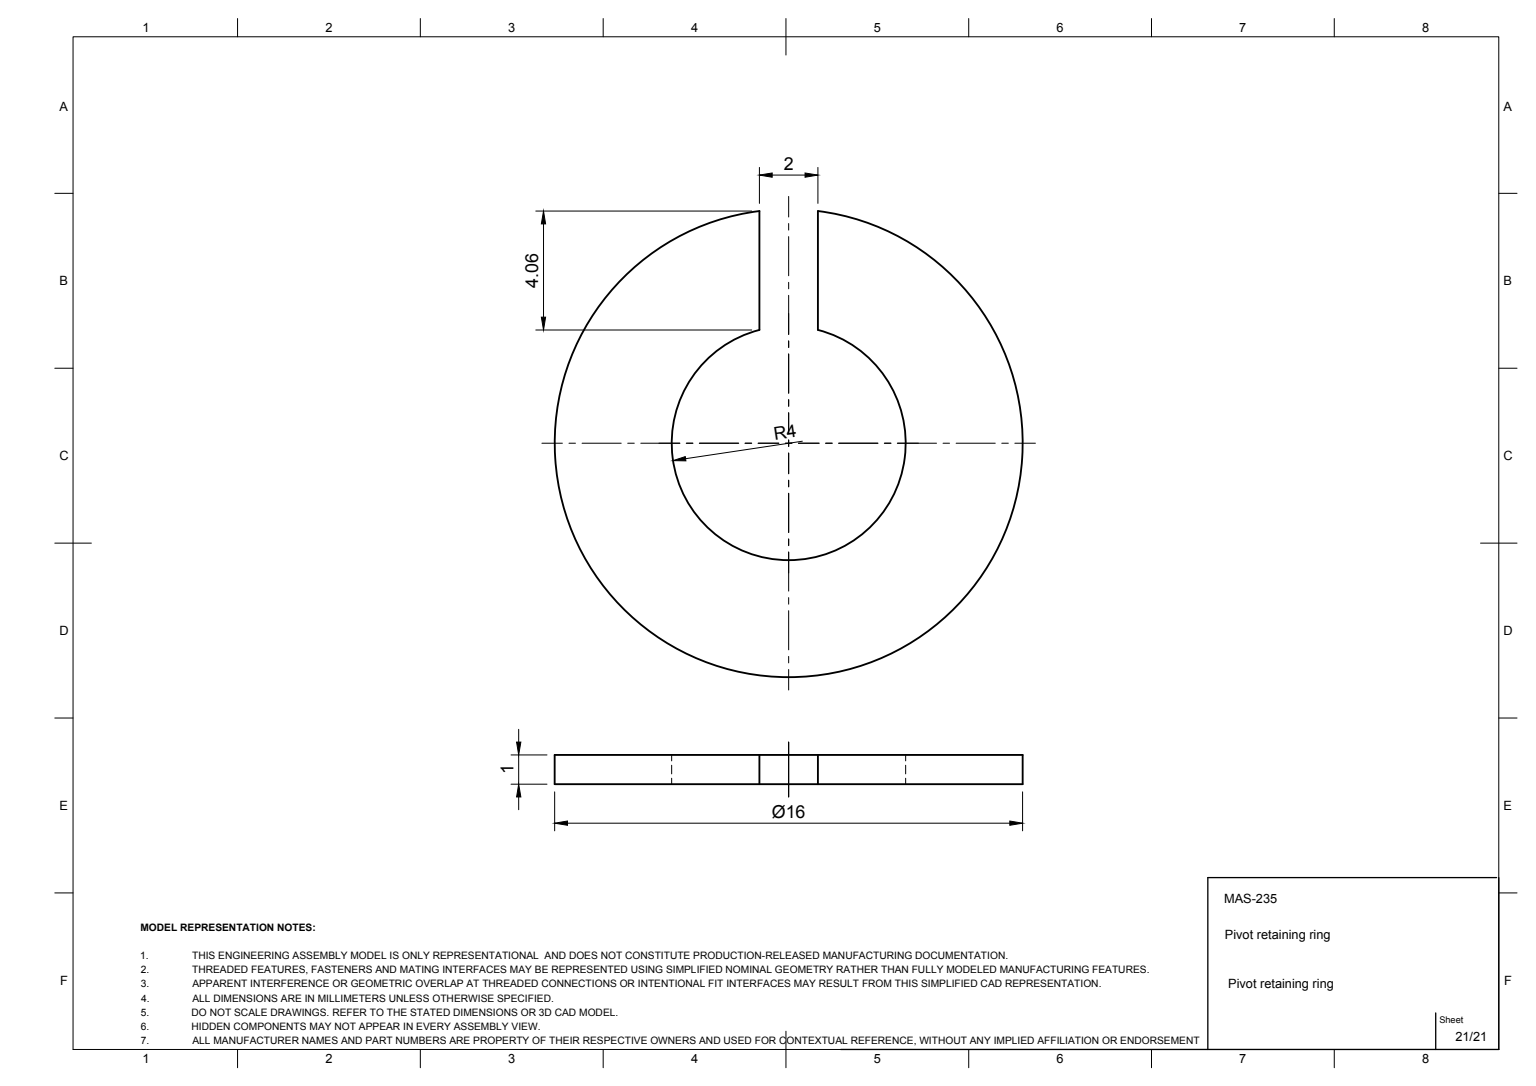
ISO-10303-21;
HEADER;
/* Generated by software containing ST-Developer
 * from STEP Tools, Inc. (www.steptools.com) 
 */

FILE_DESCRIPTION(
/* description */ ('Independent Whitworth quick-return mechanism. Crank radius40, ground-
center spacing80, lever180, connecting rod160, output guide X200. Nomi
nal stroke180 and long/short phase ratio2. Retained guide rods, replac
eable bearing sleeves and captured sliding shoe. No load or production
 rating assigned.'),
/* implementation_level */ '2;1');

FILE_NAME(
/* name */ 'Pivot retaining ring.step',
/* time_stamp */ '2026-11-09T18:22:56-08:00',
/* author */ (''),
/* organization */ (''),
/* preprocessor_version */ 'ST-DEVELOPER v20.2',
/* originating_system */ 'Autodesk Translation Framework v15.17.0.0',
/* authorisation */ '');

FILE_SCHEMA (('AUTOMOTIVE_DESIGN { 1 0 10303 214 3 1 1 }'));
ENDSEC;

DATA;
#10=MECHANICAL_DESIGN_GEOMETRIC_PRESENTATION_REPRESENTATION('',(#238),#4388);
#198=SHAPE_REPRESENTATION_RELATIONSHIP('SRR','None',#4497,#218);
#218=ADVANCED_BREP_SHAPE_REPRESENTATION('',(#258),#4387);
#238=STYLED_ITEM('',(#4599),#258);
#258=MANIFOLD_SOLID_BREP('Body1',#2343);
#401=PLANE('',#2845);
#402=PLANE('',#2846);
#403=PLANE('',#2847);
#404=PLANE('',#2854);
#546=FACE_OUTER_BOUND('',#753,.T.);
#547=FACE_OUTER_BOUND('',#754,.T.);
#548=FACE_OUTER_BOUND('',#755,.T.);
#549=FACE_OUTER_BOUND('',#756,.T.);
#550=FACE_OUTER_BOUND('',#757,.T.);
#551=FACE_OUTER_BOUND('',#758,.T.);
#753=EDGE_LOOP('',(#2092,#2093,#2094,#2095));
#754=EDGE_LOOP('',(#2096,#2097,#2098,#2099));
#755=EDGE_LOOP('',(#2100,#2101,#2102,#2103));
#756=EDGE_LOOP('',(#2104,#2105,#2106,#2107));
#757=EDGE_LOOP('',(#2108,#2109,#2110,#2111));
#758=EDGE_LOOP('',(#2112,#2113,#2114,#2115));
#890=LINE('',#4280,#1029);
#891=LINE('',#4282,#1030);
#892=LINE('',#4284,#1031);
#893=LINE('',#4285,#1032);
#894=LINE('',#4289,#1033);
#895=LINE('',#4291,#1034);
#896=LINE('',#4293,#1035);
#897=LINE('',#4294,#1036);
#1029=VECTOR('',#3590,10.);
#1030=VECTOR('',#3591,10.);
#1031=VECTOR('',#3592,10.);
#1032=VECTOR('',#3593,10.);
#1033=VECTOR('',#3596,10.);
#1034=VECTOR('',#3597,10.);
#1035=VECTOR('',#3598,10.);
#1036=VECTOR('',#3599,10.);
#1155=CIRCLE('',#2848,8.);
#1156=CIRCLE('',#2849,4.);
#1157=CIRCLE('',#2851,4.);
#1158=CIRCLE('',#2853,8.);
#1325=VERTEX_POINT('',#4278);
#1326=VERTEX_POINT('',#4279);
#1327=VERTEX_POINT('',#4281);
#1328=VERTEX_POINT('',#4283);
#1329=VERTEX_POINT('',#4287);
#1330=VERTEX_POINT('',#4288);
#1331=VERTEX_POINT('',#4290);
#1332=VERTEX_POINT('',#4292);
#1582=EDGE_CURVE('',#1325,#1326,#890,.T.);
#1583=EDGE_CURVE('',#1327,#1325,#891,.T.);
#1584=EDGE_CURVE('',#1328,#1327,#892,.T.);
#1585=EDGE_CURVE('',#1326,#1328,#893,.T.);
#1586=EDGE_CURVE('',#1329,#1330,#894,.T.);
#1587=EDGE_CURVE('',#1331,#1329,#895,.T.);
#1588=EDGE_CURVE('',#1332,#1331,#896,.T.);
#1589=EDGE_CURVE('',#1330,#1332,#897,.T.);
#1590=EDGE_CURVE('',#1327,#1332,#1155,.T.);
#1591=EDGE_CURVE('',#1330,#1325,#1156,.T.);
#1592=EDGE_CURVE('',#1329,#1326,#1157,.T.);
#1593=EDGE_CURVE('',#1328,#1331,#1158,.T.);
#2092=ORIENTED_EDGE('',*,*,#1582,.F.);
#2093=ORIENTED_EDGE('',*,*,#1583,.F.);
#2094=ORIENTED_EDGE('',*,*,#1584,.F.);
#2095=ORIENTED_EDGE('',*,*,#1585,.F.);
#2096=ORIENTED_EDGE('',*,*,#1586,.F.);
#2097=ORIENTED_EDGE('',*,*,#1587,.F.);
#2098=ORIENTED_EDGE('',*,*,#1588,.F.);
#2099=ORIENTED_EDGE('',*,*,#1589,.F.);
#2100=ORIENTED_EDGE('',*,*,#1589,.T.);
#2101=ORIENTED_EDGE('',*,*,#1590,.F.);
#2102=ORIENTED_EDGE('',*,*,#1583,.T.);
#2103=ORIENTED_EDGE('',*,*,#1591,.F.);
#2104=ORIENTED_EDGE('',*,*,#1586,.T.);
#2105=ORIENTED_EDGE('',*,*,#1591,.T.);
#2106=ORIENTED_EDGE('',*,*,#1582,.T.);
#2107=ORIENTED_EDGE('',*,*,#1592,.F.);
#2108=ORIENTED_EDGE('',*,*,#1588,.T.);
#2109=ORIENTED_EDGE('',*,*,#1593,.F.);
#2110=ORIENTED_EDGE('',*,*,#1584,.T.);
#2111=ORIENTED_EDGE('',*,*,#1590,.T.);
#2112=ORIENTED_EDGE('',*,*,#1587,.T.);
#2113=ORIENTED_EDGE('',*,*,#1592,.T.);
#2114=ORIENTED_EDGE('',*,*,#1585,.T.);
#2115=ORIENTED_EDGE('',*,*,#1593,.T.);
#2175=CYLINDRICAL_SURFACE('',#2850,4.);
#2176=CYLINDRICAL_SURFACE('',#2852,8.);
#2318=ADVANCED_FACE('',(#546),#401,.F.);
#2319=ADVANCED_FACE('',(#547),#402,.F.);
#2320=ADVANCED_FACE('',(#548),#403,.F.);
#2321=ADVANCED_FACE('',(#549),#2175,.F.);
#2322=ADVANCED_FACE('',(#550),#2176,.T.);
#2323=ADVANCED_FACE('',(#551),#404,.T.);
#2343=CLOSED_SHELL('',(#2318,#2319,#2320,#2321,#2322,#2323));
#2844=AXIS2_PLACEMENT_3D('',#4276,#3586,#3587);
#2845=AXIS2_PLACEMENT_3D('',#4277,#3588,#3589);
#2846=AXIS2_PLACEMENT_3D('',#4286,#3594,#3595);
#2847=AXIS2_PLACEMENT_3D('',#4295,#3600,#3601);
#2848=AXIS2_PLACEMENT_3D('',#4296,#3602,#3603);
#2849=AXIS2_PLACEMENT_3D('',#4297,#3604,#3605);
#2850=AXIS2_PLACEMENT_3D('',#4298,#3606,#3607);
#2851=AXIS2_PLACEMENT_3D('',#4299,#3608,#3609);
#2852=AXIS2_PLACEMENT_3D('',#4300,#3610,#3611);
#2853=AXIS2_PLACEMENT_3D('',#4301,#3612,#3613);
#2854=AXIS2_PLACEMENT_3D('',#4302,#3614,#3615);
#3586=DIRECTION('axis',(0.,0.,1.));
#3587=DIRECTION('refdir',(1.,0.,0.));
#3588=DIRECTION('center_axis',(-1.,0.,0.));
#3589=DIRECTION('ref_axis',(0.,1.,0.));
#3590=DIRECTION('',(0.,0.,1.));
#3591=DIRECTION('',(0.,-1.,0.));
#3592=DIRECTION('',(0.,0.,-1.));
#3593=DIRECTION('',(0.,1.,0.));
#3594=DIRECTION('center_axis',(1.,0.,0.));
#3595=DIRECTION('ref_axis',(0.,-1.,0.));
#3596=DIRECTION('',(0.,0.,-1.));
#3597=DIRECTION('',(0.,-1.,0.));
#3598=DIRECTION('',(0.,0.,1.));
#3599=DIRECTION('',(0.,1.,0.));
#3600=DIRECTION('center_axis',(0.,0.,1.));
#3601=DIRECTION('ref_axis',(1.,0.,0.));
#3602=DIRECTION('center_axis',(0.,0.,1.));
#3603=DIRECTION('ref_axis',(1.,0.,0.));
#3604=DIRECTION('center_axis',(0.,0.,-1.));
#3605=DIRECTION('ref_axis',(1.,0.,0.));
#3606=DIRECTION('center_axis',(0.,0.,1.));
#3607=DIRECTION('ref_axis',(6.12323399573677E-17,-1.,0.));
#3608=DIRECTION('center_axis',(0.,0.,-1.));
#3609=DIRECTION('ref_axis',(1.,0.,0.));
#3610=DIRECTION('center_axis',(0.,0.,1.));
#3611=DIRECTION('ref_axis',(6.12323399573677E-17,-1.,0.));
#3612=DIRECTION('center_axis',(0.,0.,1.));
#3613=DIRECTION('ref_axis',(1.,0.,0.));
#3614=DIRECTION('center_axis',(0.,0.,1.));
#3615=DIRECTION('ref_axis',(1.,0.,0.));
#4276=CARTESIAN_POINT('',(0.,0.,0.));
#4277=CARTESIAN_POINT('Origin',(-1.,0.,1.));
#4278=CARTESIAN_POINT('',(-1.,3.87298334620742,0.));
#4279=CARTESIAN_POINT('',(-1.,3.87298334620742,1.));
#4280=CARTESIAN_POINT('',(-1.,3.87298334620742,0.));
#4281=CARTESIAN_POINT('',(-1.,7.93725393319377,0.));
#4282=CARTESIAN_POINT('',(-1.,0.,0.));
#4283=CARTESIAN_POINT('',(-1.,7.93725393319377,1.));
#4284=CARTESIAN_POINT('',(-1.,7.93725393319377,0.));
#4285=CARTESIAN_POINT('',(-1.,0.,1.));
#4286=CARTESIAN_POINT('Origin',(1.,16.,1.));
#4287=CARTESIAN_POINT('',(1.,3.87298334620742,1.));
#4288=CARTESIAN_POINT('',(1.,3.87298334620742,0.));
#4289=CARTESIAN_POINT('',(1.,3.87298334620742,0.));
#4290=CARTESIAN_POINT('',(1.,7.93725393319377,1.));
#4291=CARTESIAN_POINT('',(1.,8.,1.));
#4292=CARTESIAN_POINT('',(1.,7.93725393319377,0.));
#4293=CARTESIAN_POINT('',(1.,7.93725393319377,0.));
#4294=CARTESIAN_POINT('',(1.,8.,0.));
#4295=CARTESIAN_POINT('Origin',(0.,0.,0.));
#4296=CARTESIAN_POINT('Origin',(0.,0.,0.));
#4297=CARTESIAN_POINT('Origin',(0.,0.,0.));
#4298=CARTESIAN_POINT('Origin',(0.,0.,0.));
#4299=CARTESIAN_POINT('Origin',(0.,0.,1.));
#4300=CARTESIAN_POINT('Origin',(0.,0.,0.));
#4301=CARTESIAN_POINT('Origin',(0.,0.,1.));
#4302=CARTESIAN_POINT('Origin',(0.,0.,1.));
#4365=UNCERTAINTY_MEASURE_WITH_UNIT(LENGTH_MEASURE(0.01),#4389,
'DISTANCE_ACCURACY_VALUE',
'Maximum model space distance between geometric entities at asserted c
onnectivities');
#4366=UNCERTAINTY_MEASURE_WITH_UNIT(LENGTH_MEASURE(0.01),#4389,
'DISTANCE_ACCURACY_VALUE',
'Maximum model space distance between geometric entities at asserted c
onnectivities');
#4387=(
GEOMETRIC_REPRESENTATION_CONTEXT(3)
GLOBAL_UNCERTAINTY_ASSIGNED_CONTEXT((#4365))
GLOBAL_UNIT_ASSIGNED_CONTEXT((#4389,#4391,#4392))
REPRESENTATION_CONTEXT('','3D')
);
#4388=(
GEOMETRIC_REPRESENTATION_CONTEXT(3)
GLOBAL_UNCERTAINTY_ASSIGNED_CONTEXT((#4366))
GLOBAL_UNIT_ASSIGNED_CONTEXT((#4389,#4391,#4392))
REPRESENTATION_CONTEXT('','3D')
);
#4389=(
LENGTH_UNIT()
NAMED_UNIT(*)
SI_UNIT(.MILLI.,.METRE.)
);
#4391=(
NAMED_UNIT(*)
PLANE_ANGLE_UNIT()
SI_UNIT($,.RADIAN.)
);
#4392=(
NAMED_UNIT(*)
SI_UNIT($,.STERADIAN.)
SOLID_ANGLE_UNIT()
);
#4413=SHAPE_DEFINITION_REPRESENTATION(#4434,#4497);
#4434=PRODUCT_DEFINITION_SHAPE('',$,#4519);
#4497=SHAPE_REPRESENTATION('',(#2844),#4387);
#4498=PRODUCT_DEFINITION_CONTEXT('part definition',#4563,'design');
#4519=PRODUCT_DEFINITION('Pivot retaining ring','Pivot retaining ring',
#4540,#4498);
#4540=PRODUCT_DEFINITION_FORMATION('',$,#4585);
#4563=APPLICATION_CONTEXT(
'Core Data for Automotive Mechanical Design Process');
#4564=PRODUCT_CONTEXT('part definition',#4563,'mechanical');
#4585=PRODUCT('Pivot retaining ring','Pivot retaining ring',$,(#4564));
#4599=PRESENTATION_STYLE_ASSIGNMENT((#4613));
#4613=SURFACE_STYLE_USAGE(.BOTH.,#4627);
#4627=SURFACE_SIDE_STYLE('',(#4641));
#4641=SURFACE_STYLE_FILL_AREA(#4655);
#4655=FILL_AREA_STYLE('Dark gray',(#4669));
#4669=FILL_AREA_STYLE_COLOUR('Dark gray',#4683);
#4683=COLOUR_RGB('Dark gray',0.250980392156863,0.282352941176471,0.32156862745098);
ENDSEC;
END-ISO-10303-21;
